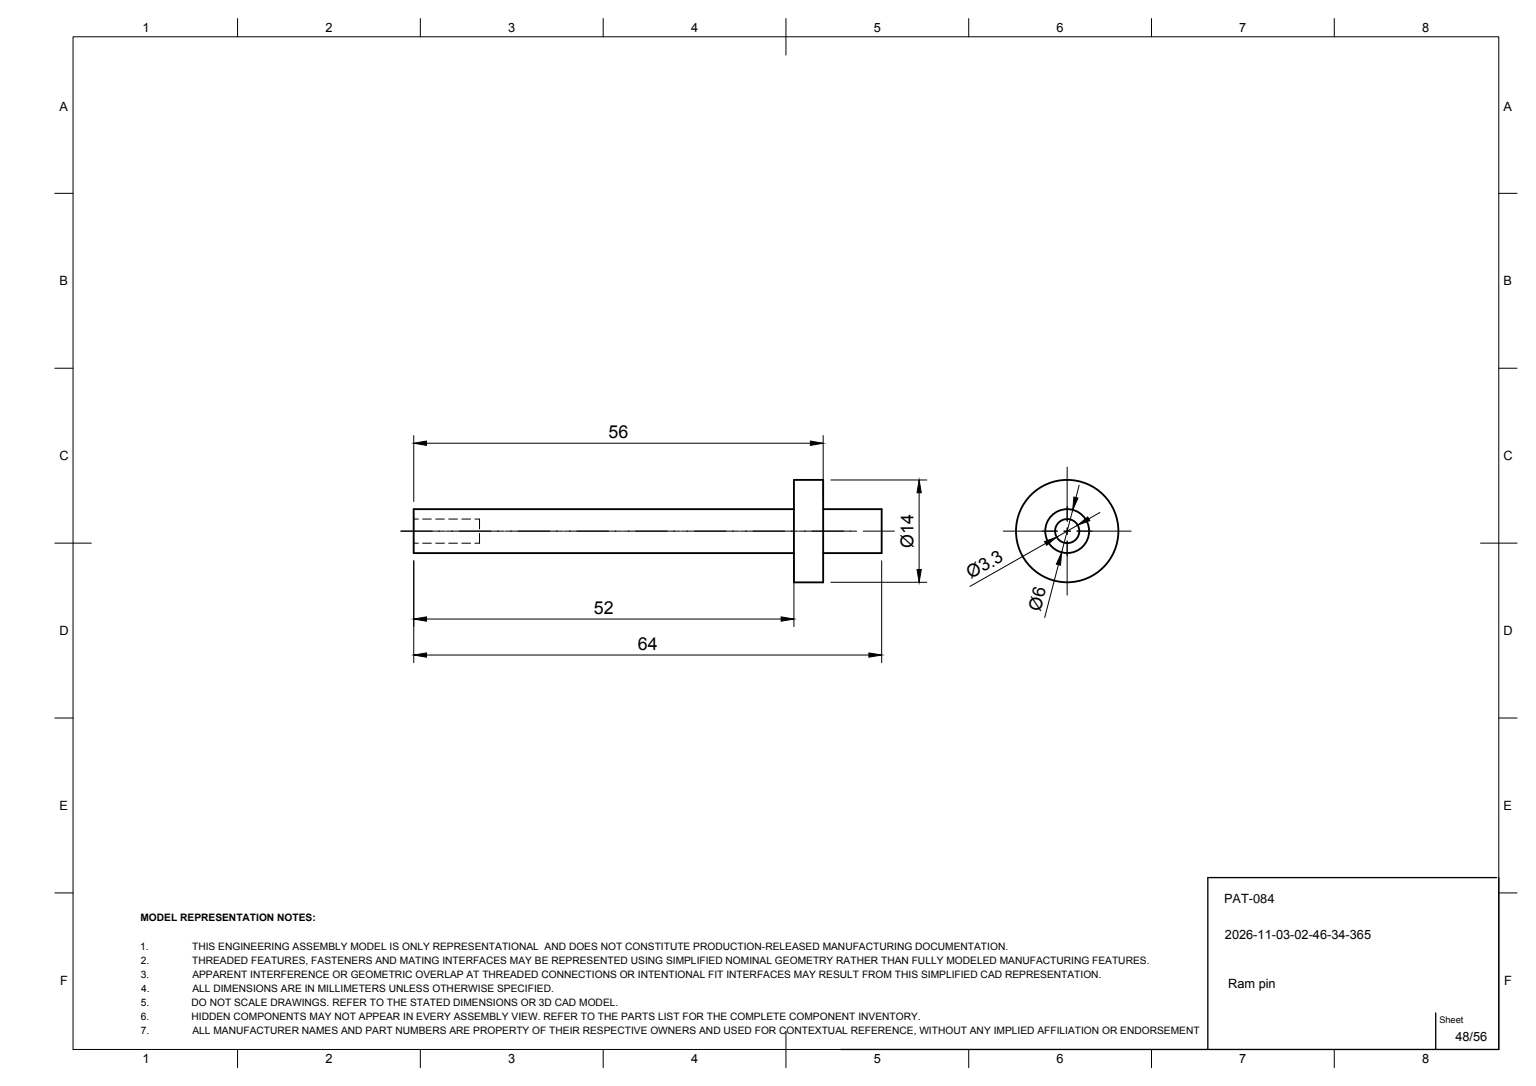
ISO-10303-21;
HEADER;
/* Generated by software containing ST-Developer
 * from STEP Tools, Inc. (www.steptools.com) 
 */

FILE_DESCRIPTION(
/* description */ ('Quick-return (Whitworth) mechanism'),
/* implementation_level */ '2;1');

FILE_NAME(
/* name */ 'Ram pin.step',
/* time_stamp */ '2026-10-28T03:25:57-07:00',
/* author */ (''),
/* organization */ (''),
/* preprocessor_version */ 'ST-DEVELOPER v20.2',
/* originating_system */ 'Autodesk Translation Framework v15.17.0.0',
/* authorisation */ '');

FILE_SCHEMA (('AUTOMOTIVE_DESIGN { 1 0 10303 214 3 1 1 }'));
ENDSEC;

DATA;
#10=MECHANICAL_DESIGN_GEOMETRIC_PRESENTATION_REPRESENTATION('',(#533),#14878);
#437=SHAPE_REPRESENTATION_RELATIONSHIP('SRR','None',#15111,#481);
#481=ADVANCED_BREP_SHAPE_REPRESENTATION('',(#584),#14868);
#533=STYLED_ITEM('',(#15406),#584);
#584=MANIFOLD_SOLID_BREP('Body1',#7888);
#767=FACE_BOUND('',#2063,.T.);
#768=FACE_BOUND('',#2065,.T.);
#769=FACE_BOUND('',#2070,.T.);
#976=PLANE('',#9176);
#977=PLANE('',#9177);
#978=PLANE('',#9180);
#979=PLANE('',#9188);
#980=PLANE('',#9189);
#1418=FACE_OUTER_BOUND('',#2060,.T.);
#1419=FACE_OUTER_BOUND('',#2061,.T.);
#1420=FACE_OUTER_BOUND('',#2062,.T.);
#1421=FACE_OUTER_BOUND('',#2064,.T.);
#1422=FACE_OUTER_BOUND('',#2066,.T.);
#1423=FACE_OUTER_BOUND('',#2067,.T.);
#1424=FACE_OUTER_BOUND('',#2068,.T.);
#1425=FACE_OUTER_BOUND('',#2069,.T.);
#1426=FACE_OUTER_BOUND('',#2071,.T.);
#2060=EDGE_LOOP('',(#6790,#6791,#6792,#6793));
#2061=EDGE_LOOP('',(#6794));
#2062=EDGE_LOOP('',(#6795));
#2063=EDGE_LOOP('',(#6796));
#2064=EDGE_LOOP('',(#6797));
#2065=EDGE_LOOP('',(#6798));
#2066=EDGE_LOOP('',(#6799,#6800,#6801,#6802));
#2067=EDGE_LOOP('',(#6803,#6804,#6805,#6806));
#2068=EDGE_LOOP('',(#6807,#6808,#6809,#6810));
#2069=EDGE_LOOP('',(#6811));
#2070=EDGE_LOOP('',(#6812));
#2071=EDGE_LOOP('',(#6813));
#2533=LINE('',#14253,#3056);
#2534=LINE('',#14267,#3057);
#2535=LINE('',#14270,#3058);
#2536=LINE('',#14275,#3059);
#3056=VECTOR('',#11342,0.164999999999999);
#3057=VECTOR('',#11361,0.699999999999999);
#3058=VECTOR('',#11364,0.300000000000001);
#3059=VECTOR('',#11371,0.300000000000001);
#3581=CIRCLE('',#9174,0.164999999999999);
#3582=CIRCLE('',#9175,0.164999999999999);
#3583=CIRCLE('',#9178,0.699999999999999);
#3584=CIRCLE('',#9179,0.300000000000001);
#3585=CIRCLE('',#9181,0.699999999999999);
#3586=CIRCLE('',#9182,0.300000000000001);
#3587=CIRCLE('',#9185,0.300000000000001);
#3588=CIRCLE('',#9187,0.300000000000001);
#4150=VERTEX_POINT('',#14250);
#4151=VERTEX_POINT('',#14252);
#4152=VERTEX_POINT('',#14257);
#4153=VERTEX_POINT('',#14259);
#4154=VERTEX_POINT('',#14262);
#4155=VERTEX_POINT('',#14264);
#4156=VERTEX_POINT('',#14269);
#4157=VERTEX_POINT('',#14273);
#5052=EDGE_CURVE('',#4150,#4150,#3581,.T.);
#5053=EDGE_CURVE('',#4150,#4151,#2533,.T.);
#5054=EDGE_CURVE('',#4151,#4151,#3582,.T.);
#5055=EDGE_CURVE('',#4152,#4152,#3583,.T.);
#5056=EDGE_CURVE('',#4153,#4153,#3584,.T.);
#5057=EDGE_CURVE('',#4154,#4154,#3585,.T.);
#5058=EDGE_CURVE('',#4155,#4155,#3586,.T.);
#5059=EDGE_CURVE('',#4152,#4154,#2534,.T.);
#5060=EDGE_CURVE('',#4155,#4156,#2535,.T.);
#5061=EDGE_CURVE('',#4156,#4156,#3587,.T.);
#5062=EDGE_CURVE('',#4157,#4157,#3588,.T.);
#5063=EDGE_CURVE('',#4157,#4153,#2536,.T.);
#6790=ORIENTED_EDGE('',*,*,#5052,.F.);
#6791=ORIENTED_EDGE('',*,*,#5053,.T.);
#6792=ORIENTED_EDGE('',*,*,#5054,.F.);
#6793=ORIENTED_EDGE('',*,*,#5053,.F.);
#6794=ORIENTED_EDGE('',*,*,#5052,.T.);
#6795=ORIENTED_EDGE('',*,*,#5055,.T.);
#6796=ORIENTED_EDGE('',*,*,#5056,.F.);
#6797=ORIENTED_EDGE('',*,*,#5057,.F.);
#6798=ORIENTED_EDGE('',*,*,#5058,.F.);
#6799=ORIENTED_EDGE('',*,*,#5055,.F.);
#6800=ORIENTED_EDGE('',*,*,#5059,.T.);
#6801=ORIENTED_EDGE('',*,*,#5057,.T.);
#6802=ORIENTED_EDGE('',*,*,#5059,.F.);
#6803=ORIENTED_EDGE('',*,*,#5058,.T.);
#6804=ORIENTED_EDGE('',*,*,#5060,.T.);
#6805=ORIENTED_EDGE('',*,*,#5061,.T.);
#6806=ORIENTED_EDGE('',*,*,#5060,.F.);
#6807=ORIENTED_EDGE('',*,*,#5062,.F.);
#6808=ORIENTED_EDGE('',*,*,#5063,.T.);
#6809=ORIENTED_EDGE('',*,*,#5056,.T.);
#6810=ORIENTED_EDGE('',*,*,#5063,.F.);
#6811=ORIENTED_EDGE('',*,*,#5062,.T.);
#6812=ORIENTED_EDGE('',*,*,#5054,.T.);
#6813=ORIENTED_EDGE('',*,*,#5061,.F.);
#7360=CYLINDRICAL_SURFACE('',#9173,0.164999999999999);
#7361=CYLINDRICAL_SURFACE('',#9183,0.699999999999999);
#7362=CYLINDRICAL_SURFACE('',#9184,0.300000000000001);
#7363=CYLINDRICAL_SURFACE('',#9186,0.300000000000001);
#7749=ADVANCED_FACE('',(#1418),#7360,.F.);
#7750=ADVANCED_FACE('',(#1419),#976,.T.);
#7751=ADVANCED_FACE('',(#1420,#767),#977,.T.);
#7752=ADVANCED_FACE('',(#1421,#768),#978,.F.);
#7753=ADVANCED_FACE('',(#1422),#7361,.T.);
#7754=ADVANCED_FACE('',(#1423),#7362,.T.);
#7755=ADVANCED_FACE('',(#1424),#7363,.T.);
#7756=ADVANCED_FACE('',(#1425,#769),#979,.T.);
#7757=ADVANCED_FACE('',(#1426),#980,.F.);
#7888=CLOSED_SHELL('',(#7749,#7750,#7751,#7752,#7753,#7754,#7755,#7756,
#7757));
#9172=AXIS2_PLACEMENT_3D('',#14248,#11336,#11337);
#9173=AXIS2_PLACEMENT_3D('',#14249,#11338,#11339);
#9174=AXIS2_PLACEMENT_3D('',#14251,#11340,#11341);
#9175=AXIS2_PLACEMENT_3D('',#14254,#11343,#11344);
#9176=AXIS2_PLACEMENT_3D('',#14255,#11345,#11346);
#9177=AXIS2_PLACEMENT_3D('',#14256,#11347,#11348);
#9178=AXIS2_PLACEMENT_3D('',#14258,#11349,#11350);
#9179=AXIS2_PLACEMENT_3D('',#14260,#11351,#11352);
#9180=AXIS2_PLACEMENT_3D('',#14261,#11353,#11354);
#9181=AXIS2_PLACEMENT_3D('',#14263,#11355,#11356);
#9182=AXIS2_PLACEMENT_3D('',#14265,#11357,#11358);
#9183=AXIS2_PLACEMENT_3D('',#14266,#11359,#11360);
#9184=AXIS2_PLACEMENT_3D('',#14268,#11362,#11363);
#9185=AXIS2_PLACEMENT_3D('',#14271,#11365,#11366);
#9186=AXIS2_PLACEMENT_3D('',#14272,#11367,#11368);
#9187=AXIS2_PLACEMENT_3D('',#14274,#11369,#11370);
#9188=AXIS2_PLACEMENT_3D('',#14276,#11372,#11373);
#9189=AXIS2_PLACEMENT_3D('',#14277,#11374,#11375);
#11336=DIRECTION('axis',(0.,0.,1.));
#11337=DIRECTION('refdir',(1.,0.,0.));
#11338=DIRECTION('center_axis',(0.,0.,1.));
#11339=DIRECTION('ref_axis',(1.,0.,0.));
#11340=DIRECTION('center_axis',(0.,0.,1.));
#11341=DIRECTION('ref_axis',(1.,0.,0.));
#11342=DIRECTION('',(0.,0.,1.));
#11343=DIRECTION('center_axis',(0.,0.,-1.));
#11344=DIRECTION('ref_axis',(1.,0.,0.));
#11345=DIRECTION('center_axis',(0.,0.,1.));
#11346=DIRECTION('ref_axis',(1.,0.,0.));
#11347=DIRECTION('center_axis',(0.,0.,1.));
#11348=DIRECTION('ref_axis',(1.,0.,0.));
#11349=DIRECTION('center_axis',(0.,0.,1.));
#11350=DIRECTION('ref_axis',(1.,0.,0.));
#11351=DIRECTION('center_axis',(0.,0.,1.));
#11352=DIRECTION('ref_axis',(1.,0.,0.));
#11353=DIRECTION('center_axis',(0.,0.,1.));
#11354=DIRECTION('ref_axis',(1.,0.,0.));
#11355=DIRECTION('center_axis',(0.,0.,1.));
#11356=DIRECTION('ref_axis',(1.,0.,0.));
#11357=DIRECTION('center_axis',(0.,0.,-1.));
#11358=DIRECTION('ref_axis',(1.,0.,0.));
#11359=DIRECTION('center_axis',(0.,0.,1.));
#11360=DIRECTION('ref_axis',(1.,0.,0.));
#11361=DIRECTION('',(0.,0.,-1.));
#11362=DIRECTION('center_axis',(0.,0.,1.));
#11363=DIRECTION('ref_axis',(1.,0.,0.));
#11364=DIRECTION('',(0.,0.,-1.));
#11365=DIRECTION('center_axis',(0.,0.,1.));
#11366=DIRECTION('ref_axis',(1.,0.,0.));
#11367=DIRECTION('center_axis',(0.,0.,1.));
#11368=DIRECTION('ref_axis',(1.,0.,0.));
#11369=DIRECTION('center_axis',(0.,0.,1.));
#11370=DIRECTION('ref_axis',(1.,0.,0.));
#11371=DIRECTION('',(0.,0.,-1.));
#11372=DIRECTION('center_axis',(0.,0.,1.));
#11373=DIRECTION('ref_axis',(1.,0.,0.));
#11374=DIRECTION('center_axis',(0.,0.,1.));
#11375=DIRECTION('ref_axis',(1.,0.,0.));
#14248=CARTESIAN_POINT('',(0.,0.,0.));
#14249=CARTESIAN_POINT('Origin',(9.16515138991168,16.,8.9));
#14250=CARTESIAN_POINT('',(9.00015138991168,16.,8.9));
#14251=CARTESIAN_POINT('Origin',(9.16515138991168,16.,8.9));
#14252=CARTESIAN_POINT('',(9.00015138991168,16.,9.8));
#14253=CARTESIAN_POINT('',(9.00015138991168,16.,8.9));
#14254=CARTESIAN_POINT('Origin',(9.16515138991168,16.,9.8));
#14255=CARTESIAN_POINT('Origin',(9.16515138991168,16.,8.9));
#14256=CARTESIAN_POINT('Origin',(9.16515138991168,16.,4.6));
#14257=CARTESIAN_POINT('',(8.46515138991168,16.,4.6));
#14258=CARTESIAN_POINT('Origin',(9.16515138991168,16.,4.6));
#14259=CARTESIAN_POINT('',(8.86515138991168,16.,4.6));
#14260=CARTESIAN_POINT('Origin',(9.16515138991168,16.,4.6));
#14261=CARTESIAN_POINT('Origin',(9.16515138991168,16.,4.2));
#14262=CARTESIAN_POINT('',(8.46515138991168,16.,4.2));
#14263=CARTESIAN_POINT('Origin',(9.16515138991168,16.,4.2));
#14264=CARTESIAN_POINT('',(8.86515138991168,16.,4.2));
#14265=CARTESIAN_POINT('Origin',(9.16515138991168,16.,4.2));
#14266=CARTESIAN_POINT('Origin',(9.16515138991168,16.,4.2));
#14267=CARTESIAN_POINT('',(8.46515138991168,16.,4.2));
#14268=CARTESIAN_POINT('Origin',(9.16515138991168,16.,3.4));
#14269=CARTESIAN_POINT('',(8.86515138991168,16.,3.4));
#14270=CARTESIAN_POINT('',(8.86515138991168,16.,3.4));
#14271=CARTESIAN_POINT('Origin',(9.16515138991168,16.,3.4));
#14272=CARTESIAN_POINT('Origin',(9.16515138991168,16.,3.4));
#14273=CARTESIAN_POINT('',(8.86515138991168,16.,9.8));
#14274=CARTESIAN_POINT('Origin',(9.16515138991168,16.,9.8));
#14275=CARTESIAN_POINT('',(8.86515138991168,16.,3.4));
#14276=CARTESIAN_POINT('Origin',(9.16515138991168,16.,9.8));
#14277=CARTESIAN_POINT('Origin',(9.16515138991168,16.,3.4));
#14814=UNCERTAINTY_MEASURE_WITH_UNIT(LENGTH_MEASURE(0.001),#14879,
'DISTANCE_ACCURACY_VALUE',
'Maximum model space distance between geometric entities at asserted c
onnectivities');
#14824=UNCERTAINTY_MEASURE_WITH_UNIT(LENGTH_MEASURE(0.001),#14879,
'DISTANCE_ACCURACY_VALUE',
'Maximum model space distance between geometric entities at asserted c
onnectivities');
#14868=(
GEOMETRIC_REPRESENTATION_CONTEXT(3)
GLOBAL_UNCERTAINTY_ASSIGNED_CONTEXT((#14814))
GLOBAL_UNIT_ASSIGNED_CONTEXT((#14879,#14881,#14882))
REPRESENTATION_CONTEXT('','3D')
);
#14878=(
GEOMETRIC_REPRESENTATION_CONTEXT(3)
GLOBAL_UNCERTAINTY_ASSIGNED_CONTEXT((#14824))
GLOBAL_UNIT_ASSIGNED_CONTEXT((#14879,#14881,#14882))
REPRESENTATION_CONTEXT('','3D')
);
#14879=(
LENGTH_UNIT()
NAMED_UNIT(*)
SI_UNIT(.CENTI.,.METRE.)
);
#14881=(
NAMED_UNIT(*)
PLANE_ANGLE_UNIT()
SI_UNIT($,.RADIAN.)
);
#14882=(
NAMED_UNIT(*)
SI_UNIT($,.STERADIAN.)
SOLID_ANGLE_UNIT()
);
#14926=SHAPE_DEFINITION_REPRESENTATION(#14988,#15111);
#14988=PRODUCT_DEFINITION_SHAPE('',$,#15165);
#15111=SHAPE_REPRESENTATION('',(#9172),#14868);
#15121=PRODUCT_DEFINITION_CONTEXT('part definition',#15282,'design');
#15165=PRODUCT_DEFINITION('Ram pin','Ram pin',#15218,#15121);
#15218=PRODUCT_DEFINITION_FORMATION('',$,#15327);
#15282=APPLICATION_CONTEXT(
'Core Data for Automotive Mechanical Design Process');
#15283=PRODUCT_CONTEXT('part definition',#15282,'mechanical');
#15327=PRODUCT('Ram pin','Ram pin','Ram pin',(#15283));
#15400=COLOUR_RGB('Grey',0.48,0.52,0.57);
#15401=FILL_AREA_STYLE_COLOUR('',#15400);
#15402=FILL_AREA_STYLE('',(#15401));
#15403=SURFACE_STYLE_FILL_AREA(#15402);
#15404=SURFACE_SIDE_STYLE('',(#15403));
#15405=SURFACE_STYLE_USAGE(.BOTH.,#15404);
#15406=PRESENTATION_STYLE_ASSIGNMENT((#15405));
ENDSEC;
END-ISO-10303-21;
